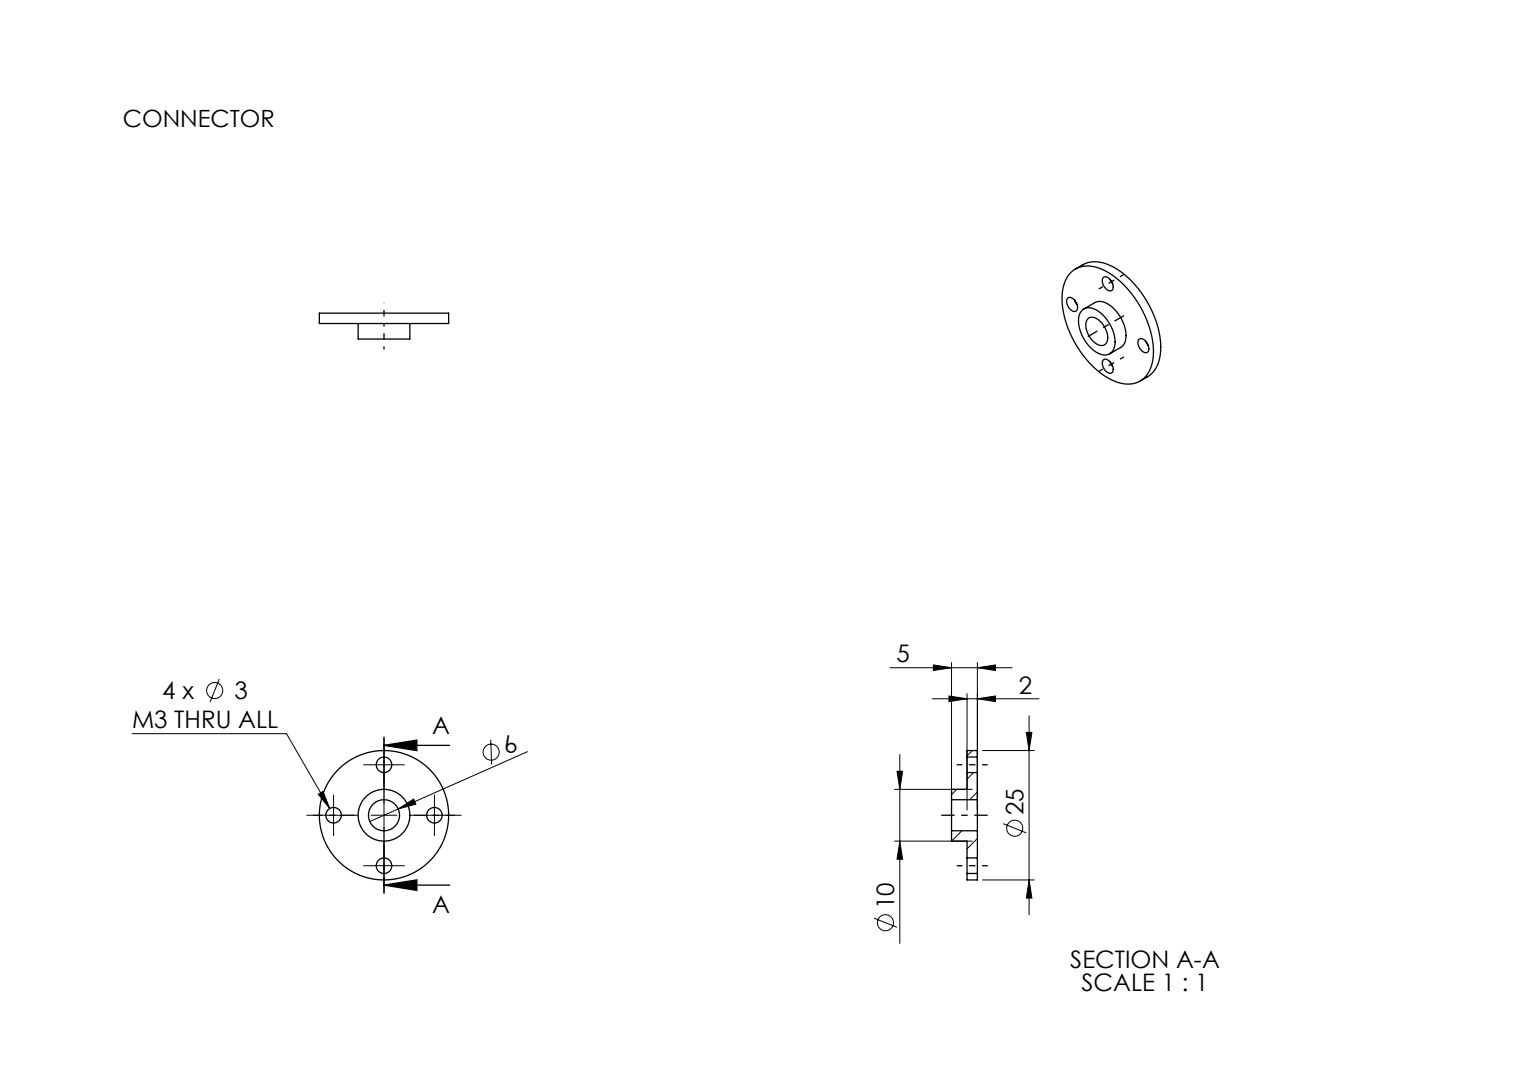
ISO-10303-21;
HEADER;
FILE_DESCRIPTION (('STEP AP214'),
    '1' );
FILE_NAME ('connector.step',
    '2026-10-04T10:31:01',
    ( '' ),
    ( '' ),
    'SwSTEP 2.0',
    'SolidWorks 2026',
    '' );
FILE_SCHEMA (( 'AUTOMOTIVE_DESIGN' ));
ENDSEC;

DATA;
#41=FACE_BOUND ( 'NONE', #6027, .T. ) ;
#54=DIRECTION ( 'NONE',  ( 0.000000000000000000, 0.000000000000000000, 1.000000000000000000 ) ) ;
#65=DIRECTION ( 'NONE',  ( 1.000000000000000000, 0.000000000000000000, 0.000000000000000000 ) ) ;
#67=ORIENTED_EDGE ( 'NONE', *, *, #457, .F. ) ;
#77=LINE ( 'NONE', #5895, #15592 ) ;
#103=EDGE_LOOP ( 'NONE', ( #8397, #1444 ) ) ;
#146=LINE ( 'NONE', #13353, #5536 ) ;
#156=CARTESIAN_POINT ( 'NONE',  ( 12.50000000000000533, 1.530808498934192113E-15, 0.000000000000000000 ) ) ;
#162=ORIENTED_EDGE ( 'NONE', *, *, #10171, .F. ) ;
#176=CARTESIAN_POINT ( 'NONE',  ( 0.000000000000000000, 0.000000000000000000, 5.000000000000004441 ) ) ;
#183=LINE ( 'NONE', #11083, #4538 ) ;
#188=DIRECTION ( 'NONE',  ( 0.000000000000000000, 0.000000000000000000, 1.000000000000000000 ) ) ;
#206=CARTESIAN_POINT ( 'NONE',  ( -12.50000000000000533, 0.000000000000000000, 2.000000000000001776 ) ) ;
#218=DIRECTION ( 'NONE',  ( 0.000000000000000000, 0.000000000000000000, -1.000000000000000000 ) ) ;
#226=EDGE_LOOP ( 'NONE', ( #14083, #11757, #15041, #247 ) ) ;
#228=CARTESIAN_POINT ( 'NONE',  ( -11.25000000000000355, 3.419666426228851687E-14, 2.000000000000001776 ) ) ;
#239=ORIENTED_EDGE ( 'NONE', *, *, #1750, .T. ) ;
#247=ORIENTED_EDGE ( 'NONE', *, *, #524, .F. ) ;
#282=CARTESIAN_POINT ( 'NONE',  ( 1.500000000000000000, -9.750000000000003553, 2.000000000000001776 ) ) ;
#288=( NAMED_UNIT ( * ) SI_UNIT ( $, .STERADIAN. ) SOLID_ANGLE_UNIT ( ) );
#297=CYLINDRICAL_SURFACE ( 'NONE', #14167, 1.499999999999999556 ) ;
#304=DIRECTION ( 'NONE',  ( 0.000000000000000000, 0.000000000000000000, 1.000000000000000000 ) ) ;
#319=DIRECTION ( 'NONE',  ( 1.000000000000000000, 0.000000000000000000, 0.000000000000000000 ) ) ;
#393=DIRECTION ( 'NONE',  ( 1.000000000000000000, 0.000000000000000000, 0.000000000000000000 ) ) ;
#402=DIRECTION ( 'NONE',  ( 1.000000000000000000, 0.000000000000000000, 0.000000000000000000 ) ) ;
#409=DIRECTION ( 'NONE',  ( 1.000000000000000000, 0.000000000000000000, 0.000000000000000000 ) ) ;
#435=DIRECTION ( 'NONE',  ( 0.000000000000000000, 0.000000000000000000, -1.000000000000000000 ) ) ;
#440=LINE ( 'NONE', #9200, #5916 ) ;
#446=AXIS2_PLACEMENT_3D ( 'NONE', #11551, #13858, #6488 ) ;
#457=EDGE_CURVE ( 'NONE', #15709, #6637, #10482, .T. ) ;
#482=CARTESIAN_POINT ( 'NONE',  ( -9.750000000000003553, 3.401296724241641415E-14, 2.000000000000001776 ) ) ;
#486=DIRECTION ( 'NONE',  ( 0.000000000000000000, 0.000000000000000000, 1.000000000000000000 ) ) ;
#495=ORIENTED_EDGE ( 'NONE', *, *, #4351, .F. ) ;
#512=VERTEX_POINT ( 'NONE', #14445 ) ;
#524=EDGE_CURVE ( 'NONE', #8787, #10326, #14889, .T. ) ;
#532=ORIENTED_EDGE ( 'NONE', *, *, #10481, .F. ) ;
#594=EDGE_CURVE ( 'NONE', #12272, #12484, #3857, .T. ) ;
#639=EDGE_CURVE ( 'NONE', #1178, #15136, #14644, .T. ) ;
#670=DIRECTION ( 'NONE',  ( 0.000000000000000000, 0.000000000000000000, 1.000000000000000000 ) ) ;
#775=( LENGTH_UNIT ( ) NAMED_UNIT ( * ) SI_UNIT ( .MILLI., .METRE. ) );
#788=EDGE_CURVE ( 'NONE', #5458, #12720, #7023, .T. ) ;
#816=AXIS2_PLACEMENT_3D ( 'NONE', #2518, #3778, #4670 ) ;
#859=LINE ( 'NONE', #9458, #13806 ) ;
#878=VERTEX_POINT ( 'NONE', #12172 ) ;
#897=MECHANICAL_DESIGN_GEOMETRIC_PRESENTATION_REPRESENTATION('',(#8272),#8792);
#904=UNCERTAINTY_MEASURE_WITH_UNIT (LENGTH_MEASURE( 1.000000000000000082E-05 ), #8679, 'distance_accuracy_value', 'NONE');
#920=VERTEX_POINT ( 'NONE', #156 ) ;
#1053=LINE ( 'NONE', #4803, #11886 ) ;
#1080=AXIS2_PLACEMENT_3D ( 'NONE', #13512, #14641, #13442 ) ;
#1118=ORIENTED_EDGE ( 'NONE', *, *, #11482, .T. ) ;
#1133=VERTEX_POINT ( 'NONE', #11682 ) ;
#1140=FACE_BOUND ( 'NONE', #7178, .T. ) ;
#1145=DIRECTION ( 'NONE',  ( -1.000000000000000000, 0.000000000000000000, 0.000000000000000000 ) ) ;
#1152=DIRECTION ( 'NONE',  ( 1.000000000000000000, 0.000000000000000000, 0.000000000000000000 ) ) ;
#1178=VERTEX_POINT ( 'NONE', #15425 ) ;
#1194=ORIENTED_EDGE ( 'NONE', *, *, #6676, .T. ) ;
#1209=CARTESIAN_POINT ( 'NONE',  ( 12.50000000000000533, 1.530808498934192113E-15, 2.000000000000001776 ) ) ;
#1213=CIRCLE ( 'NONE', #1462, 3.000000000000000000 ) ;
#1248=DIRECTION ( 'NONE',  ( 0.000000000000000000, 0.000000000000000000, 1.000000000000000000 ) ) ;
#1265=CARTESIAN_POINT ( 'NONE',  ( -2.897581130414634077E-17, 9.750000000000003553, 2.000000000000001776 ) ) ;
#1294=DIRECTION ( 'NONE',  ( 0.000000000000000000, 0.000000000000000000, 1.000000000000000000 ) ) ;
#1338=CIRCLE ( 'NONE', #13277, 1.500000000000000000 ) ;
#1378=CARTESIAN_POINT ( 'NONE',  ( 0.000000000000000000, 0.000000000000000000, 2.000000000000001776 ) ) ;
#1432=EDGE_CURVE ( 'NONE', #878, #13950, #13112, .T. ) ;
#1444=ORIENTED_EDGE ( 'NONE', *, *, #13970, .F. ) ;
#1462=AXIS2_PLACEMENT_3D ( 'NONE', #1507, #11295, #393 ) ;
#1468=CARTESIAN_POINT ( 'NONE',  ( 2.897581130414634077E-17, -9.750000000000003553, 2.000000000000001776 ) ) ;
#1507=CARTESIAN_POINT ( 'NONE',  ( 0.000000000000000000, 0.000000000000000000, 5.000000000000004441 ) ) ;
#1511=FACE_OUTER_BOUND ( 'NONE', #12331, .T. ) ;
#1519=ADVANCED_FACE ( 'NONE', ( #3542, #41 ), #8413, .T. ) ;
#1586=ORIENTED_EDGE ( 'NONE', *, *, #13291, .F. ) ;
#1622=ADVANCED_FACE ( 'NONE', ( #14135 ), #15187, .T. ) ;
#1637=AXIS2_PLACEMENT_3D ( 'NONE', #11385, #486, #15285 ) ;
#1651=DIRECTION ( 'NONE',  ( 1.000000000000000000, 0.000000000000000000, 0.000000000000000000 ) ) ;
#1740=ORIENTED_EDGE ( 'NONE', *, *, #8830, .T. ) ;
#1750=EDGE_CURVE ( 'NONE', #2410, #3136, #2201, .T. ) ;
#1778=ORIENTED_EDGE ( 'NONE', *, *, #13016, .T. ) ;
#1814=FACE_OUTER_BOUND ( 'NONE', #10483, .T. ) ;
#1823=ADVANCED_FACE ( 'NONE', ( #12301 ), #7614, .T. ) ;
#1834=CIRCLE ( 'NONE', #816, 1.500000000000000000 ) ;
#1847=CIRCLE ( 'NONE', #2630, 1.499999999999999556 ) ;
#1882=CYLINDRICAL_SURFACE ( 'NONE', #12144, 1.499999999999999556 ) ;
#1887=DIRECTION ( 'NONE',  ( 0.000000000000000000, 0.000000000000000000, -1.000000000000000000 ) ) ;
#1891=DIRECTION ( 'NONE',  ( 0.000000000000000000, 0.000000000000000000, 1.000000000000000000 ) ) ;
#1957=ORIENTED_EDGE ( 'NONE', *, *, #12525, .T. ) ;
#1972=CIRCLE ( 'NONE', #6060, 5.000000000000000000 ) ;
#1974=AXIS2_PLACEMENT_3D ( 'NONE', #8448, #2622, #7478 ) ;
#2004=EDGE_CURVE ( 'NONE', #15509, #10326, #146, .T. ) ;
#2114=ORIENTED_EDGE ( 'NONE', *, *, #11739, .F. ) ;
#2117=DIRECTION ( 'NONE',  ( 0.000000000000000000, 0.000000000000000000, 1.000000000000000000 ) ) ;
#2137=CARTESIAN_POINT ( 'NONE',  ( -5.000000000000000000, 0.000000000000000000, 2.000000000000001776 ) ) ;
#2149=EDGE_CURVE ( 'NONE', #12720, #2410, #13507, .T. ) ;
#2195=EDGE_CURVE ( 'NONE', #9577, #3564, #5089, .T. ) ;
#2201=CIRCLE ( 'NONE', #15686, 1.499999999999999556 ) ;
#2304=CYLINDRICAL_SURFACE ( 'NONE', #13300, 1.500000000000000000 ) ;
#2333=UNCERTAINTY_MEASURE_WITH_UNIT (LENGTH_MEASURE( 1.000000000000000082E-05 ), #8736, 'distance_accuracy_value', 'NONE');
#2352=LINE ( 'NONE', #14611, #7682 ) ;
#2398=CIRCLE ( 'NONE', #5980, 5.000000000000000000 ) ;
#2410=VERTEX_POINT ( 'NONE', #7285 ) ;
#2425=AXIS2_PLACEMENT_3D ( 'NONE', #10542, #15483, #4496 ) ;
#2429=VERTEX_POINT ( 'NONE', #11011 ) ;
#2442=SHAPE_REPRESENTATION_RELATIONSHIP ( 'NONE' , 'NONE' ,  #3660, #4613 ) ;
#2498=EDGE_CURVE ( 'NONE', #3136, #2410, #6811, .T. ) ;
#2504=CYLINDRICAL_SURFACE ( 'NONE', #14010, 3.000000000000000000 ) ;
#2518=CARTESIAN_POINT ( 'NONE',  ( -2.897581130414634077E-17, 9.750000000000003553, 0.000000000000000000 ) ) ;
#2550=CARTESIAN_POINT ( 'NONE',  ( -9.750000000000003553, 3.401296724241641415E-14, 0.000000000000000000 ) ) ;
#2577=DIRECTION ( 'NONE',  ( 0.000000000000000000, 0.000000000000000000, -1.000000000000000000 ) ) ;
#2599=CARTESIAN_POINT ( 'NONE',  ( 0.000000000000000000, 0.000000000000000000, 5.000000000000004441 ) ) ;
#2622=DIRECTION ( 'NONE',  ( 0.000000000000000000, 0.000000000000000000, 1.000000000000000000 ) ) ;
#2630=AXIS2_PLACEMENT_3D ( 'NONE', #6474, #15129, #11308 ) ;
#2651=EDGE_CURVE ( 'NONE', #9577, #15709, #4254, .T. ) ;
#2672=DIRECTION ( 'NONE',  ( 0.000000000000000000, 0.000000000000000000, 1.000000000000000000 ) ) ;
#2747=AXIS2_PLACEMENT_3D ( 'NONE', #6769, #14144, #10650 ) ;
#2770=AXIS2_PLACEMENT_3D ( 'NONE', #176, #10049, #409 ) ;
#2777=FACE_BOUND ( 'NONE', #103, .T. ) ;
#2789=MECHANICAL_DESIGN_GEOMETRIC_PRESENTATION_REPRESENTATION('',(#4319),#14743);
#2919=VECTOR ( 'NONE', #8245, 1000.000000000000000 ) ;
#2952=AXIS2_PLACEMENT_3D ( 'NONE', #2550, #14647, #10822 ) ;
#2974=DIRECTION ( 'NONE',  ( 0.000000000000000000, 0.000000000000000000, 1.000000000000000000 ) ) ;
#3004=AXIS2_PLACEMENT_3D ( 'NONE', #12157, #11913, #65 ) ;
#3039=AXIS2_PLACEMENT_3D ( 'NONE', #6856, #13626, #10063 ) ;
#3044=ORIENTED_EDGE ( 'NONE', *, *, #9648, .F. ) ;
#3074=PRODUCT_DEFINITION_CONTEXT ( 'detailed design', #12070, 'design' ) ;
#3125=FACE_OUTER_BOUND ( 'NONE', #13175, .T. ) ;
#3136=VERTEX_POINT ( 'NONE', #8994 ) ;
#3210=ORIENTED_EDGE ( 'NONE', *, *, #1750, .F. ) ;
#3267=ADVANCED_FACE ( 'NONE', ( #12778 ), #1882, .F. ) ;
#3289=ORIENTED_EDGE ( 'NONE', *, *, #8249, .F. ) ;
#3347=ORIENTED_EDGE ( 'NONE', *, *, #11780, .F. ) ;
#3377=CARTESIAN_POINT ( 'NONE',  ( 12.50000000000000533, 1.530808498934192113E-15, 2.000000000000001776 ) ) ;
#3455=DIRECTION ( 'NONE',  ( 0.000000000000000000, 0.000000000000000000, 1.000000000000000000 ) ) ;
#3542=FACE_OUTER_BOUND ( 'NONE', #14730, .T. ) ;
#3556=COLOUR_RGB ( '', 0.40784314, 0.44705882, 0.49803922) ;
#3564=VERTEX_POINT ( 'NONE', #2137 ) ;
#3585=EDGE_LOOP ( 'NONE', ( #9691, #5379, #12917, #11080 ) ) ;
#3587=ORIENTED_EDGE ( 'NONE', *, *, #7892, .T. ) ;
#3599=ORIENTED_EDGE ( 'NONE', *, *, #2498, .T. ) ;
#3660=SHAPE_REPRESENTATION ( 'connector', ( #14201 ), #13708 ) ;
#3680=ORIENTED_EDGE ( 'NONE', *, *, #788, .F. ) ;
#3706=VECTOR ( 'NONE', #435, 1000.000000000000000 ) ;
#3710=FILL_AREA_STYLE ('',( #11189 ) ) ;
#3721=CARTESIAN_POINT ( 'NONE',  ( 8.250000000000003553, -1.019131563299854308E-13, 2.000000000000001776 ) ) ;
#3750=CARTESIAN_POINT ( 'NONE',  ( 9.750000000000003553, -1.020968533498575335E-13, 0.000000000000000000 ) ) ;
#3767=CARTESIAN_POINT ( 'NONE',  ( 5.000000000000000000, 6.123233995736766282E-16, 2.000000000000001776 ) ) ;
#3778=DIRECTION ( 'NONE',  ( 0.000000000000000000, 0.000000000000000000, 1.000000000000000000 ) ) ;
#3780=DIRECTION ( 'NONE',  ( 0.000000000000000000, 0.000000000000000000, -1.000000000000000000 ) ) ;
#3806=PRESENTATION_STYLE_ASSIGNMENT (( #7165 ) ) ;
#3809=FACE_BOUND ( 'NONE', #5043, .T. ) ;
#3814=ADVANCED_FACE ( 'NONE', ( #13359 ), #7401, .F. ) ;
#3834=ORIENTED_EDGE ( 'NONE', *, *, #11087, .T. ) ;
#3854=ADVANCED_FACE ( 'NONE', ( #12087 ), #11133, .F. ) ;
#3857=LINE ( 'NONE', #206, #3706 ) ;
#3859=CIRCLE ( 'NONE', #5903, 12.50000000000000533 ) ;
#3878=CIRCLE ( 'NONE', #10488, 1.500000000000000000 ) ;
#3882=FACE_BOUND ( 'NONE', #7908, .T. ) ;
#3911=ORIENTED_EDGE ( 'NONE', *, *, #13470, .F. ) ;
#3971=ORIENTED_EDGE ( 'NONE', *, *, #8593, .F. ) ;
#4015=DIRECTION ( 'NONE',  ( 1.000000000000000000, 0.000000000000000000, 0.000000000000000000 ) ) ;
#4146=DIRECTION ( 'NONE',  ( 1.000000000000000000, 0.000000000000000000, 0.000000000000000000 ) ) ;
#4237=EDGE_CURVE ( 'NONE', #7182, #15136, #1053, .T. ) ;
#4254=CIRCLE ( 'NONE', #9097, 5.000000000000000000 ) ;
#4312=AXIS2_PLACEMENT_3D ( 'NONE', #9668, #14509, #7041 ) ;
#4319=STYLED_ITEM ( 'NONE', ( #11033 ), #4613 ) ;
#4322=AXIS2_PLACEMENT_3D ( 'NONE', #10172, #10019, #14866 ) ;
#4334=ORIENTED_EDGE ( 'NONE', *, *, #2149, .T. ) ;
#4351=EDGE_CURVE ( 'NONE', #8237, #15509, #14960, .T. ) ;
#4388=CARTESIAN_POINT ( 'NONE',  ( -2.897581130414634077E-17, 9.750000000000003553, 0.000000000000000000 ) ) ;
#4419=EDGE_LOOP ( 'NONE', ( #8309, #10379, #12079, #7755 ) ) ;
#4474=DIRECTION ( 'NONE',  ( 0.000000000000000000, 0.000000000000000000, -1.000000000000000000 ) ) ;
#4496=DIRECTION ( 'NONE',  ( 1.000000000000000000, 0.000000000000000000, 0.000000000000000000 ) ) ;
#4538=VECTOR ( 'NONE', #1294, 1000.000000000000000 ) ;
#4567=CARTESIAN_POINT ( 'NONE',  ( -12.50000000000000533, 0.000000000000000000, 2.000000000000001776 ) ) ;
#4613=ADVANCED_BREP_SHAPE_REPRESENTATION ( '', ( #10345, #14201 ), #13708 ) ;
#4614=CARTESIAN_POINT ( 'NONE',  ( 0.000000000000000000, 0.000000000000000000, 5.000000000000004441 ) ) ;
#4634=CARTESIAN_POINT ( 'NONE',  ( 0.000000000000000000, 0.000000000000000000, 5.000000000000004441 ) ) ;
#4667=CARTESIAN_POINT ( 'NONE',  ( -11.25000000000000355, 3.419666426228851687E-14, 0.000000000000000000 ) ) ;
#4670=DIRECTION ( 'NONE',  ( 1.000000000000000000, 0.000000000000000000, 0.000000000000000000 ) ) ;
#4727=EDGE_LOOP ( 'NONE', ( #6809, #1118 ) ) ;
#4738=CARTESIAN_POINT ( 'NONE',  ( 0.000000000000000000, 0.000000000000000000, 2.000000000000001776 ) ) ;
#4771=PRODUCT_DEFINITION_FORMATION_WITH_SPECIFIED_SOURCE ( 'ANY', '', #12844, .NOT_KNOWN. ) ;
#4803=CARTESIAN_POINT ( 'NONE',  ( 1.500000000000000000, -9.750000000000003553, 2.000000000000001776 ) ) ;
#4813=PLANE ( 'NONE',  #4312 ) ;
#4840=SURFACE_STYLE_FILL_AREA ( #3710 ) ;
#4849=ADVANCED_FACE ( 'NONE', ( #8400, #1140, #4894, #6005, #1511, #10848 ), #4813, .F. ) ;
#4858=FILL_AREA_STYLE ('',( #13278 ) ) ;
#4894=FACE_BOUND ( 'NONE', #4727, .T. ) ;
#4910=ORIENTED_EDGE ( 'NONE', *, *, #8830, .F. ) ;
#4913=DIRECTION ( 'NONE',  ( 0.000000000000000000, 0.000000000000000000, 1.000000000000000000 ) ) ;
#5003=ORIENTED_EDGE ( 'NONE', *, *, #8249, .T. ) ;
#5022=ORIENTED_EDGE ( 'NONE', *, *, #594, .T. ) ;
#5043=EDGE_LOOP ( 'NONE', ( #14358, #3210 ) ) ;
#5089=LINE ( 'NONE', #10174, #11620 ) ;
#5197=ORIENTED_EDGE ( 'NONE', *, *, #10481, .T. ) ;
#5221=EDGE_CURVE ( 'NONE', #8237, #8787, #8440, .T. ) ;
#5315=LINE ( 'NONE', #11420, #7927 ) ;
#5340=EDGE_LOOP ( 'NONE', ( #4910, #5511, #14806, #14609 ) ) ;
#5372=ADVANCED_FACE ( 'NONE', ( #6447 ), #15178, .F. ) ;
#5379=ORIENTED_EDGE ( 'NONE', *, *, #14202, .T. ) ;
#5458=VERTEX_POINT ( 'NONE', #7932 ) ;
#5460=CIRCLE ( 'NONE', #5707, 1.499999999999999556 ) ;
#5493=DIRECTION ( 'NONE',  ( 0.000000000000000000, 0.000000000000000000, -1.000000000000000000 ) ) ;
#5511=ORIENTED_EDGE ( 'NONE', *, *, #7181, .F. ) ;
#5536=VECTOR ( 'NONE', #15673, 1000.000000000000000 ) ;
#5558=ORIENTED_EDGE ( 'NONE', *, *, #5221, .T. ) ;
#5676=CARTESIAN_POINT ( 'NONE',  ( 0.000000000000000000, 0.000000000000000000, 2.000000000000001776 ) ) ;
#5707=AXIS2_PLACEMENT_3D ( 'NONE', #12298, #54, #9776 ) ;
#5727=ORIENTED_EDGE ( 'NONE', *, *, #7781, .T. ) ;
#5738=AXIS2_PLACEMENT_3D ( 'NONE', #8418, #4913, #7447 ) ;
#5838=DIRECTION ( 'NONE',  ( 0.000000000000000000, 0.000000000000000000, 1.000000000000000000 ) ) ;
#5881=CARTESIAN_POINT ( 'NONE',  ( -5.000000000000000000, 0.000000000000000000, 5.000000000000004441 ) ) ;
#5895=CARTESIAN_POINT ( 'NONE',  ( -1.500000000000000000, 9.750000000000003553, 2.000000000000001776 ) ) ;
#5903=AXIS2_PLACEMENT_3D ( 'NONE', #1378, #188, #14431 ) ;
#5916=VECTOR ( 'NONE', #670, 1000.000000000000000 ) ;
#5980=AXIS2_PLACEMENT_3D ( 'NONE', #4614, #9549, #13111 ) ;
#6005=FACE_BOUND ( 'NONE', #7392, .T. ) ;
#6023=ORIENTED_EDGE ( 'NONE', *, *, #4237, .T. ) ;
#6027=EDGE_LOOP ( 'NONE', ( #15025, #495 ) ) ;
#6060=AXIS2_PLACEMENT_3D ( 'NONE', #14965, #9956, #319 ) ;
#6063=DIRECTION ( 'NONE',  ( 0.000000000000000000, 0.000000000000000000, 1.000000000000000000 ) ) ;
#6123=DIRECTION ( 'NONE',  ( 1.000000000000000000, 0.000000000000000000, 0.000000000000000000 ) ) ;
#6136=CARTESIAN_POINT ( 'NONE',  ( -3.000000000000000000, 0.000000000000000000, 0.000000000000000000 ) ) ;
#6151=EDGE_LOOP ( 'NONE', ( #9273, #1194 ) ) ;
#6214=SURFACE_SIDE_STYLE ('',( #11128 ) ) ;
#6227=AXIS2_PLACEMENT_3D ( 'NONE', #9435, #9280, #14267 ) ;
#6290=FACE_OUTER_BOUND ( 'NONE', #6151, .T. ) ;
#6407=ORIENTED_EDGE ( 'NONE', *, *, #2149, .F. ) ;
#6442=DIRECTION ( 'NONE',  ( 0.000000000000000000, 0.000000000000000000, 1.000000000000000000 ) ) ;
#6447=FACE_OUTER_BOUND ( 'NONE', #3585, .T. ) ;
#6474=CARTESIAN_POINT ( 'NONE',  ( 9.750000000000003553, -1.020968533498575335E-13, 2.000000000000001776 ) ) ;
#6488=DIRECTION ( 'NONE',  ( 1.000000000000000000, 0.000000000000000000, 0.000000000000000000 ) ) ;
#6518=DIRECTION ( 'NONE',  ( 1.000000000000000000, 0.000000000000000000, 0.000000000000000000 ) ) ;
#6599=ADVANCED_FACE ( 'NONE', ( #10936 ), #2504, .F. ) ;
#6637=VERTEX_POINT ( 'NONE', #3767 ) ;
#6651=ADVANCED_FACE ( 'NONE', ( #13475 ), #10778, .T. ) ;
#6676=EDGE_CURVE ( 'NONE', #12347, #12272, #3859, .T. ) ;
#6680=CARTESIAN_POINT ( 'NONE',  ( 0.000000000000000000, 0.000000000000000000, 0.000000000000000000 ) ) ;
#6693=AXIS2_PLACEMENT_3D ( 'NONE', #3750, #8701, #13534 ) ;
#6705=DIRECTION ( 'NONE',  ( 0.000000000000000000, 0.000000000000000000, 1.000000000000000000 ) ) ;
#6722=CARTESIAN_POINT ( 'NONE',  ( 2.897581130414634077E-17, -9.750000000000003553, 2.000000000000001776 ) ) ;
#6757=DIRECTION ( 'NONE',  ( 1.000000000000000000, 0.000000000000000000, 0.000000000000000000 ) ) ;
#6769=CARTESIAN_POINT ( 'NONE',  ( 0.000000000000000000, 0.000000000000000000, 0.000000000000000000 ) ) ;
#6774=AXIS2_PLACEMENT_3D ( 'NONE', #1468, #2672, #4015 ) ;
#6780=CARTESIAN_POINT ( 'NONE',  ( 3.000000000000000000, 3.673940397442059868E-16, 0.000000000000000000 ) ) ;
#6806=ORIENTED_EDGE ( 'NONE', *, *, #7218, .T. ) ;
#6809=ORIENTED_EDGE ( 'NONE', *, *, #8294, .T. ) ;
#6811=CIRCLE ( 'NONE', #446, 1.499999999999999556 ) ;
#6823=AXIS2_PLACEMENT_3D ( 'NONE', #1265, #9637, #12322 ) ;
#6825=CARTESIAN_POINT ( 'NONE',  ( -2.897581130414634077E-17, 9.750000000000003553, 2.000000000000001776 ) ) ;
#6826=ADVANCED_FACE ( 'NONE', ( #9013 ), #10197, .F. ) ;
#6856=CARTESIAN_POINT ( 'NONE',  ( -2.897581130414634077E-17, 9.750000000000003553, 2.000000000000001776 ) ) ;
#6904=DIRECTION ( 'NONE',  ( 1.000000000000000000, 0.000000000000000000, 0.000000000000000000 ) ) ;
#6943=ORIENTED_EDGE ( 'NONE', *, *, #788, .T. ) ;
#6951=CYLINDRICAL_SURFACE ( 'NONE', #11523, 3.000000000000000000 ) ;
#6981=CIRCLE ( 'NONE', #6227, 1.500000000000000000 ) ;
#7023=CIRCLE ( 'NONE', #2952, 1.499999999999999556 ) ;
#7041=DIRECTION ( 'NONE',  ( 1.000000000000000000, 0.000000000000000000, 0.000000000000000000 ) ) ;
#7081=ADVANCED_FACE ( 'NONE', ( #8202, #2777, #14721, #3809, #6290, #3882 ), #8682, .T. ) ;
#7115=ORIENTED_EDGE ( 'NONE', *, *, #11087, .F. ) ;
#7119=ORIENTED_EDGE ( 'NONE', *, *, #8294, .F. ) ;
#7165=SURFACE_STYLE_USAGE ( .BOTH. , #6214 ) ;
#7178=EDGE_LOOP ( 'NONE', ( #12111, #3834 ) ) ;
#7181=EDGE_CURVE ( 'NONE', #10893, #512, #1834, .T. ) ;
#7182=VERTEX_POINT ( 'NONE', #11892 ) ;
#7199=ORIENTED_EDGE ( 'NONE', *, *, #2651, .T. ) ;
#7218=EDGE_CURVE ( 'NONE', #2429, #13435, #2352, .T. ) ;
#7277=EDGE_LOOP ( 'NONE', ( #3289, #14486 ) ) ;
#7285=CARTESIAN_POINT ( 'NONE',  ( -11.25000000000000355, 3.419666426228851687E-14, 2.000000000000001776 ) ) ;
#7305=SURFACE_STYLE_USAGE ( .BOTH. , #9925 ) ;
#7309=CARTESIAN_POINT ( 'NONE',  ( -9.750000000000003553, 3.401296724241641415E-14, 2.000000000000001776 ) ) ;
#7392=EDGE_LOOP ( 'NONE', ( #6943, #8269 ) ) ;
#7401=CYLINDRICAL_SURFACE ( 'NONE', #6823, 1.500000000000000000 ) ;
#7411=ORIENTED_EDGE ( 'NONE', *, *, #594, .F. ) ;
#7426=ORIENTED_EDGE ( 'NONE', *, *, #2195, .T. ) ;
#7434=CARTESIAN_POINT ( 'NONE',  ( 0.000000000000000000, 0.000000000000000000, 5.000000000000004441 ) ) ;
#7445=DIRECTION ( 'NONE',  ( 0.000000000000000000, 0.000000000000000000, 1.000000000000000000 ) ) ;
#7447=DIRECTION ( 'NONE',  ( 1.000000000000000000, 0.000000000000000000, 0.000000000000000000 ) ) ;
#7478=DIRECTION ( 'NONE',  ( 1.000000000000000000, 0.000000000000000000, 0.000000000000000000 ) ) ;
#7486=EDGE_LOOP ( 'NONE', ( #14634, #15623 ) ) ;
#7614=CYLINDRICAL_SURFACE ( 'NONE', #8062, 5.000000000000000000 ) ;
#7624=ORIENTED_EDGE ( 'NONE', *, *, #8678, .T. ) ;
#7682=VECTOR ( 'NONE', #14689, 1000.000000000000000 ) ;
#7755=ORIENTED_EDGE ( 'NONE', *, *, #2195, .F. ) ;
#7756=CARTESIAN_POINT ( 'NONE',  ( -1.500000000000000000, 9.750000000000003553, 2.000000000000001776 ) ) ;
#7767=CIRCLE ( 'NONE', #2425, 3.000000000000000000 ) ;
#7781=EDGE_CURVE ( 'NONE', #5458, #3136, #440, .T. ) ;
#7791=ORIENTED_EDGE ( 'NONE', *, *, #13123, .T. ) ;
#7851=EDGE_CURVE ( 'NONE', #8910, #1133, #5315, .T. ) ;
#7892=EDGE_CURVE ( 'NONE', #920, #12484, #12002, .T. ) ;
#7908=EDGE_LOOP ( 'NONE', ( #10647, #3911 ) ) ;
#7927=VECTOR ( 'NONE', #10160, 1000.000000000000000 ) ;
#7932=CARTESIAN_POINT ( 'NONE',  ( -8.250000000000003553, 3.401296724241641415E-14, 0.000000000000000000 ) ) ;
#8040=CYLINDRICAL_SURFACE ( 'NONE', #3039, 1.500000000000000000 ) ;
#8049=EDGE_LOOP ( 'NONE', ( #9978, #7119, #6023, #5003 ) ) ;
#8062=AXIS2_PLACEMENT_3D ( 'NONE', #2599, #218, #13496 ) ;
#8202=FACE_BOUND ( 'NONE', #14381, .T. ) ;
#8237=VERTEX_POINT ( 'NONE', #13862 ) ;
#8245=DIRECTION ( 'NONE',  ( 0.000000000000000000, 0.000000000000000000, -1.000000000000000000 ) ) ;
#8249=EDGE_CURVE ( 'NONE', #15136, #1178, #3878, .T. ) ;
#8269=ORIENTED_EDGE ( 'NONE', *, *, #10673, .T. ) ;
#8272=STYLED_ITEM ( 'NONE', ( #3806 ), #10345 ) ;
#8294=EDGE_CURVE ( 'NONE', #7182, #14655, #1338, .T. ) ;
#8309=ORIENTED_EDGE ( 'NONE', *, *, #12525, .F. ) ;
#8333=EDGE_LOOP ( 'NONE', ( #15336, #4334, #239, #15665 ) ) ;
#8354=AXIS2_PLACEMENT_3D ( 'NONE', #9997, #7445, #12289 ) ;
#8397=ORIENTED_EDGE ( 'NONE', *, *, #8678, .F. ) ;
#8400=FACE_BOUND ( 'NONE', #7486, .T. ) ;
#8404=UNCERTAINTY_MEASURE_WITH_UNIT (LENGTH_MEASURE( 1.000000000000000082E-05 ), #775, 'distance_accuracy_value', 'NONE');
#8413=PLANE ( 'NONE',  #14136 ) ;
#8418=CARTESIAN_POINT ( 'NONE',  ( 0.000000000000000000, 0.000000000000000000, 0.000000000000000000 ) ) ;
#8440=LINE ( 'NONE', #9711, #12943 ) ;
#8448=CARTESIAN_POINT ( 'NONE',  ( 9.750000000000003553, -1.020968533498575335E-13, 2.000000000000001776 ) ) ;
#8458=AXIS2_PLACEMENT_3D ( 'NONE', #482, #11380, #402 ) ;
#8509=( NAMED_UNIT ( * ) PLANE_ANGLE_UNIT ( ) SI_UNIT ( $, .RADIAN. ) );
#8522=CIRCLE ( 'NONE', #1637, 1.500000000000000000 ) ;
#8593=EDGE_CURVE ( 'NONE', #8910, #2429, #11502, .T. ) ;
#8678=EDGE_CURVE ( 'NONE', #1133, #13435, #1847, .T. ) ;
#8679=( LENGTH_UNIT ( ) NAMED_UNIT ( * ) SI_UNIT ( .MILLI., .METRE. ) );
#8682=PLANE ( 'NONE',  #1080 ) ;
#8701=DIRECTION ( 'NONE',  ( 0.000000000000000000, 0.000000000000000000, 1.000000000000000000 ) ) ;
#8736=( LENGTH_UNIT ( ) NAMED_UNIT ( * ) SI_UNIT ( .MILLI., .METRE. ) );
#8749=AXIS2_PLACEMENT_3D ( 'NONE', #8761, #5493, #13594 ) ;
#8761=CARTESIAN_POINT ( 'NONE',  ( 0.000000000000000000, 0.000000000000000000, 5.000000000000004441 ) ) ;
#8769=EDGE_LOOP ( 'NONE', ( #7115, #6806, #11599, #10192 ) ) ;
#8787=VERTEX_POINT ( 'NONE', #6780 ) ;
#8792=( GEOMETRIC_REPRESENTATION_CONTEXT ( 3 ) GLOBAL_UNCERTAINTY_ASSIGNED_CONTEXT ( ( #904 ) ) GLOBAL_UNIT_ASSIGNED_CONTEXT ( ( #8679, #12317, #12082 ) ) REPRESENTATION_CONTEXT ( 'NONE', 'WORKASPACE' ) );
#8797=FACE_OUTER_BOUND ( 'NONE', #15211, .T. ) ;
#8830=EDGE_CURVE ( 'NONE', #512, #13950, #77, .T. ) ;
#8910=VERTEX_POINT ( 'NONE', #14726 ) ;
#8993=DIRECTION ( 'NONE',  ( 0.000000000000000000, 0.000000000000000000, -1.000000000000000000 ) ) ;
#8994=CARTESIAN_POINT ( 'NONE',  ( -8.250000000000003553, 3.401296724241641415E-14, 2.000000000000001776 ) ) ;
#9007=ORIENTED_EDGE ( 'NONE', *, *, #11780, .T. ) ;
#9013=FACE_OUTER_BOUND ( 'NONE', #8333, .T. ) ;
#9097=AXIS2_PLACEMENT_3D ( 'NONE', #14657, #9807, #9651 ) ;
#9200=CARTESIAN_POINT ( 'NONE',  ( -8.250000000000003553, 3.401296724241641415E-14, 2.000000000000001776 ) ) ;
#9224=CARTESIAN_POINT ( 'NONE',  ( 0.000000000000000000, 0.000000000000000000, 2.000000000000001776 ) ) ;
#9273=ORIENTED_EDGE ( 'NONE', *, *, #10171, .T. ) ;
#9280=DIRECTION ( 'NONE',  ( 0.000000000000000000, 0.000000000000000000, 1.000000000000000000 ) ) ;
#9294=CARTESIAN_POINT ( 'NONE',  ( 1.500000000000000000, 9.750000000000003553, 0.000000000000000000 ) ) ;
#9328=DIRECTION ( 'NONE',  ( -1.000000000000000000, 0.000000000000000000, 0.000000000000000000 ) ) ;
#9338=ADVANCED_FACE ( 'NONE', ( #11058 ), #2304, .F. ) ;
#9366=ORIENTED_EDGE ( 'NONE', *, *, #7892, .F. ) ;
#9435=CARTESIAN_POINT ( 'NONE',  ( 2.897581130414634077E-17, -9.750000000000003553, 0.000000000000000000 ) ) ;
#9458=CARTESIAN_POINT ( 'NONE',  ( 1.500000000000000000, 9.750000000000003553, 2.000000000000001776 ) ) ;
#9461=ADVANCED_FACE ( 'NONE', ( #1814 ), #10105, .T. ) ;
#9549=DIRECTION ( 'NONE',  ( 0.000000000000000000, 0.000000000000000000, 1.000000000000000000 ) ) ;
#9577=VERTEX_POINT ( 'NONE', #5881 ) ;
#9637=DIRECTION ( 'NONE',  ( 0.000000000000000000, 0.000000000000000000, 1.000000000000000000 ) ) ;
#9645=APPLICATION_CONTEXT ( 'automotive_design' ) ;
#9648=EDGE_CURVE ( 'NONE', #10893, #878, #859, .T. ) ;
#9651=DIRECTION ( 'NONE',  ( 1.000000000000000000, 0.000000000000000000, 0.000000000000000000 ) ) ;
#9663=ORIENTED_EDGE ( 'NONE', *, *, #524, .T. ) ;
#9668=CARTESIAN_POINT ( 'NONE',  ( 0.000000000000000000, 0.000000000000000000, 0.000000000000000000 ) ) ;
#9675=DIRECTION ( 'NONE',  ( 0.000000000000000000, 0.000000000000000000, -1.000000000000000000 ) ) ;
#9691=ORIENTED_EDGE ( 'NONE', *, *, #11482, .F. ) ;
#9697=( NAMED_UNIT ( * ) PLANE_ANGLE_UNIT ( ) SI_UNIT ( $, .RADIAN. ) );
#9711=CARTESIAN_POINT ( 'NONE',  ( 3.000000000000000000, 3.673940397442059868E-16, 5.000000000000004441 ) ) ;
#9776=DIRECTION ( 'NONE',  ( 1.000000000000000000, 0.000000000000000000, 0.000000000000000000 ) ) ;
#9804=CARTESIAN_POINT ( 'NONE',  ( -1.500000000000000000, -9.750000000000003553, 0.000000000000000000 ) ) ;
#9807=DIRECTION ( 'NONE',  ( 0.000000000000000000, 0.000000000000000000, 1.000000000000000000 ) ) ;
#9876=CARTESIAN_POINT ( 'NONE',  ( 2.897581130414634077E-17, -9.750000000000003553, 2.000000000000001776 ) ) ;
#9925=SURFACE_SIDE_STYLE ('',( #4840 ) ) ;
#9956=DIRECTION ( 'NONE',  ( 0.000000000000000000, 0.000000000000000000, 1.000000000000000000 ) ) ;
#9957=EDGE_LOOP ( 'NONE', ( #10149, #162, #5022, #10281 ) ) ;
#9973=EDGE_LOOP ( 'NONE', ( #5197, #9663 ) ) ;
#9978=ORIENTED_EDGE ( 'NONE', *, *, #14202, .F. ) ;
#9997=CARTESIAN_POINT ( 'NONE',  ( 9.750000000000003553, -1.020968533498575335E-13, 2.000000000000001776 ) ) ;
#10019=DIRECTION ( 'NONE',  ( 0.000000000000000000, 0.000000000000000000, 1.000000000000000000 ) ) ;
#10049=DIRECTION ( 'NONE',  ( 0.000000000000000000, 0.000000000000000000, 1.000000000000000000 ) ) ;
#10057=AXIS2_PLACEMENT_3D ( 'NONE', #13395, #11090, #12203 ) ;
#10063=DIRECTION ( 'NONE',  ( 1.000000000000000000, 0.000000000000000000, 0.000000000000000000 ) ) ;
#10088=FACE_OUTER_BOUND ( 'NONE', #11279, .T. ) ;
#10105=CYLINDRICAL_SURFACE ( 'NONE', #8749, 5.000000000000000000 ) ;
#10149=ORIENTED_EDGE ( 'NONE', *, *, #11511, .F. ) ;
#10160=DIRECTION ( 'NONE',  ( 0.000000000000000000, 0.000000000000000000, 1.000000000000000000 ) ) ;
#10171=EDGE_CURVE ( 'NONE', #12272, #12347, #10263, .T. ) ;
#10172=CARTESIAN_POINT ( 'NONE',  ( 2.897581130414634077E-17, -9.750000000000003553, 2.000000000000001776 ) ) ;
#10174=CARTESIAN_POINT ( 'NONE',  ( -5.000000000000000000, 0.000000000000000000, 5.000000000000004441 ) ) ;
#10192=ORIENTED_EDGE ( 'NONE', *, *, #7851, .F. ) ;
#10197=CYLINDRICAL_SURFACE ( 'NONE', #8458, 1.499999999999999556 ) ;
#10212=ADVANCED_FACE ( 'NONE', ( #3125 ), #6951, .F. ) ;
#10254=CARTESIAN_POINT ( 'NONE',  ( 5.000000000000000000, 6.123233995736766282E-16, 5.000000000000004441 ) ) ;
#10263=CIRCLE ( 'NONE', #12286, 12.50000000000000533 ) ;
#10281=ORIENTED_EDGE ( 'NONE', *, *, #13291, .T. ) ;
#10290=AXIS2_PLACEMENT_3D ( 'NONE', #4388, #6705, #4146 ) ;
#10326=VERTEX_POINT ( 'NONE', #6136 ) ;
#10345=MANIFOLD_SOLID_BREP ( 'Extrude-Thin1', #14349 ) ;
#10379=ORIENTED_EDGE ( 'NONE', *, *, #457, .T. ) ;
#10481=EDGE_CURVE ( 'NONE', #10326, #8787, #7767, .T. ) ;
#10482=LINE ( 'NONE', #15335, #12335 ) ;
#10483=EDGE_LOOP ( 'NONE', ( #67, #13332, #7426, #1778 ) ) ;
#10488=AXIS2_PLACEMENT_3D ( 'NONE', #6722, #2974, #11556 ) ;
#10524=DIRECTION ( 'NONE',  ( 0.000000000000000000, 0.000000000000000000, 1.000000000000000000 ) ) ;
#10542=CARTESIAN_POINT ( 'NONE',  ( 0.000000000000000000, 0.000000000000000000, 0.000000000000000000 ) ) ;
#10544=DIRECTION ( 'NONE',  ( 1.000000000000000000, 0.000000000000000000, 0.000000000000000000 ) ) ;
#10647=ORIENTED_EDGE ( 'NONE', *, *, #13016, .F. ) ;
#10650=DIRECTION ( 'NONE',  ( 1.000000000000000000, 0.000000000000000000, 0.000000000000000000 ) ) ;
#10673=EDGE_CURVE ( 'NONE', #12720, #5458, #15130, .T. ) ;
#10681=CARTESIAN_POINT ( 'NONE',  ( 2.897581130414634077E-17, -9.750000000000003553, 0.000000000000000000 ) ) ;
#10778=CYLINDRICAL_SURFACE ( 'NONE', #12242, 12.50000000000000533 ) ;
#10822=DIRECTION ( 'NONE',  ( 1.000000000000000000, 0.000000000000000000, 0.000000000000000000 ) ) ;
#10848=FACE_BOUND ( 'NONE', #9973, .T. ) ;
#10893=VERTEX_POINT ( 'NONE', #9294 ) ;
#10908=ORIENTED_EDGE ( 'NONE', *, *, #1432, .F. ) ;
#10936=FACE_OUTER_BOUND ( 'NONE', #226, .T. ) ;
#10982=DIRECTION ( 'NONE',  ( 1.000000000000000000, 0.000000000000000000, 0.000000000000000000 ) ) ;
#11011=CARTESIAN_POINT ( 'NONE',  ( 8.250000000000003553, -1.019131563299854308E-13, 0.000000000000000000 ) ) ;
#11033=PRESENTATION_STYLE_ASSIGNMENT (( #7305 ) ) ;
#11058=FACE_OUTER_BOUND ( 'NONE', #8049, .T. ) ;
#11080=ORIENTED_EDGE ( 'NONE', *, *, #4237, .F. ) ;
#11083=CARTESIAN_POINT ( 'NONE',  ( -1.500000000000000000, -9.750000000000003553, 2.000000000000001776 ) ) ;
#11087=EDGE_CURVE ( 'NONE', #2429, #8910, #5460, .T. ) ;
#11090=DIRECTION ( 'NONE',  ( 0.000000000000000000, 0.000000000000000000, 1.000000000000000000 ) ) ;
#11128=SURFACE_STYLE_FILL_AREA ( #4858 ) ;
#11133=CYLINDRICAL_SURFACE ( 'NONE', #1974, 1.499999999999999556 ) ;
#11189=FILL_AREA_STYLE_COLOUR ( '', #3556 ) ;
#11247=AXIS2_PLACEMENT_3D ( 'NONE', #11882, #3455, #10544 ) ;
#11279=EDGE_LOOP ( 'NONE', ( #15102, #3971, #14102, #7624 ) ) ;
#11295=DIRECTION ( 'NONE',  ( 0.000000000000000000, 0.000000000000000000, 1.000000000000000000 ) ) ;
#11296=CIRCLE ( 'NONE', #10290, 1.500000000000000000 ) ;
#11308=DIRECTION ( 'NONE',  ( 1.000000000000000000, 0.000000000000000000, 0.000000000000000000 ) ) ;
#11359=AXIS2_PLACEMENT_3D ( 'NONE', #9224, #1887, #12783 ) ;
#11380=DIRECTION ( 'NONE',  ( 0.000000000000000000, 0.000000000000000000, 1.000000000000000000 ) ) ;
#11385=CARTESIAN_POINT ( 'NONE',  ( -2.897581130414634077E-17, 9.750000000000003553, 2.000000000000001776 ) ) ;
#11420=CARTESIAN_POINT ( 'NONE',  ( 11.25000000000000355, -1.020968533498575335E-13, 2.000000000000001776 ) ) ;
#11482=EDGE_CURVE ( 'NONE', #14655, #7182, #6981, .T. ) ;
#11502=CIRCLE ( 'NONE', #6693, 1.499999999999999556 ) ;
#11511=EDGE_CURVE ( 'NONE', #12347, #920, #14117, .T. ) ;
#11513=DIRECTION ( 'NONE',  ( 0.000000000000000000, 0.000000000000000000, 1.000000000000000000 ) ) ;
#11523=AXIS2_PLACEMENT_3D ( 'NONE', #4634, #4474, #9328 ) ;
#11551=CARTESIAN_POINT ( 'NONE',  ( -9.750000000000003553, 3.401296724241641415E-14, 2.000000000000001776 ) ) ;
#11556=DIRECTION ( 'NONE',  ( 1.000000000000000000, 0.000000000000000000, 0.000000000000000000 ) ) ;
#11599=ORIENTED_EDGE ( 'NONE', *, *, #13970, .T. ) ;
#11620=VECTOR ( 'NONE', #8993, 1000.000000000000000 ) ;
#11661=DIRECTION ( 'NONE',  ( 0.000000000000000000, 0.000000000000000000, 1.000000000000000000 ) ) ;
#11682=CARTESIAN_POINT ( 'NONE',  ( 11.25000000000000355, -1.020968533498575335E-13, 2.000000000000001776 ) ) ;
#11713=SHAPE_DEFINITION_REPRESENTATION ( #13501, #3660 ) ;
#11739=EDGE_CURVE ( 'NONE', #512, #10893, #11296, .T. ) ;
#11757=ORIENTED_EDGE ( 'NONE', *, *, #4351, .T. ) ;
#11780=EDGE_CURVE ( 'NONE', #13950, #878, #8522, .T. ) ;
#11855=DIRECTION ( 'NONE',  ( 1.000000000000000000, 0.000000000000000000, 0.000000000000000000 ) ) ;
#11882=CARTESIAN_POINT ( 'NONE',  ( 0.000000000000000000, 0.000000000000000000, 0.000000000000000000 ) ) ;
#11886=VECTOR ( 'NONE', #5838, 1000.000000000000000 ) ;
#11892=CARTESIAN_POINT ( 'NONE',  ( 1.500000000000000000, -9.750000000000003553, 0.000000000000000000 ) ) ;
#11913=DIRECTION ( 'NONE',  ( 0.000000000000000000, 0.000000000000000000, 1.000000000000000000 ) ) ;
#12002=CIRCLE ( 'NONE', #11247, 12.50000000000000533 ) ;
#12053=DIRECTION ( 'NONE',  ( 0.000000000000000000, 0.000000000000000000, 1.000000000000000000 ) ) ;
#12070=APPLICATION_CONTEXT ( 'automotive_design' ) ;
#12079=ORIENTED_EDGE ( 'NONE', *, *, #13470, .T. ) ;
#12082=( NAMED_UNIT ( * ) SI_UNIT ( $, .STERADIAN. ) SOLID_ANGLE_UNIT ( ) );
#12087=FACE_OUTER_BOUND ( 'NONE', #8769, .T. ) ;
#12111=ORIENTED_EDGE ( 'NONE', *, *, #8593, .T. ) ;
#12144=AXIS2_PLACEMENT_3D ( 'NONE', #15339, #2117, #6757 ) ;
#12157=CARTESIAN_POINT ( 'NONE',  ( 0.000000000000000000, 0.000000000000000000, 2.000000000000001776 ) ) ;
#12172=CARTESIAN_POINT ( 'NONE',  ( 1.500000000000000000, 9.750000000000003553, 2.000000000000001776 ) ) ;
#12203=DIRECTION ( 'NONE',  ( 1.000000000000000000, 0.000000000000000000, 0.000000000000000000 ) ) ;
#12242=AXIS2_PLACEMENT_3D ( 'NONE', #4738, #2577, #12279 ) ;
#12272=VERTEX_POINT ( 'NONE', #4567 ) ;
#12279=DIRECTION ( 'NONE',  ( -1.000000000000000000, 0.000000000000000000, 0.000000000000000000 ) ) ;
#12286=AXIS2_PLACEMENT_3D ( 'NONE', #5676, #10524, #11855 ) ;
#12289=DIRECTION ( 'NONE',  ( 1.000000000000000000, 0.000000000000000000, 0.000000000000000000 ) ) ;
#12298=CARTESIAN_POINT ( 'NONE',  ( 9.750000000000003553, -1.020968533498575335E-13, 0.000000000000000000 ) ) ;
#12301=FACE_OUTER_BOUND ( 'NONE', #4419, .T. ) ;
#12317=( NAMED_UNIT ( * ) PLANE_ANGLE_UNIT ( ) SI_UNIT ( $, .RADIAN. ) );
#12322=DIRECTION ( 'NONE',  ( 1.000000000000000000, 0.000000000000000000, 0.000000000000000000 ) ) ;
#12331=EDGE_LOOP ( 'NONE', ( #1586, #9366 ) ) ;
#12335=VECTOR ( 'NONE', #3780, 1000.000000000000000 ) ;
#12347=VERTEX_POINT ( 'NONE', #1209 ) ;
#12384=CARTESIAN_POINT ( 'NONE',  ( 9.750000000000003553, -1.020968533498575335E-13, 2.000000000000001776 ) ) ;
#12484=VERTEX_POINT ( 'NONE', #13306 ) ;
#12525=EDGE_CURVE ( 'NONE', #15709, #9577, #2398, .T. ) ;
#12537=COLOUR_RGB ( '', 0.40784314, 0.44705882, 0.49803922) ;
#12644=ADVANCED_FACE ( 'NONE', ( #10088 ), #297, .F. ) ;
#12720=VERTEX_POINT ( 'NONE', #4667 ) ;
#12778=FACE_OUTER_BOUND ( 'NONE', #13600, .T. ) ;
#12783=DIRECTION ( 'NONE',  ( -1.000000000000000000, 0.000000000000000000, 0.000000000000000000 ) ) ;
#12844=PRODUCT ( 'connector', 'connector', '', ( #14023 ) ) ;
#12917=ORIENTED_EDGE ( 'NONE', *, *, #639, .T. ) ;
#12943=VECTOR ( 'NONE', #14790, 1000.000000000000000 ) ;
#13016=EDGE_CURVE ( 'NONE', #3564, #6637, #1972, .T. ) ;
#13031=ORIENTED_EDGE ( 'NONE', *, *, #6676, .F. ) ;
#13111=DIRECTION ( 'NONE',  ( 1.000000000000000000, 0.000000000000000000, 0.000000000000000000 ) ) ;
#13112=CIRCLE ( 'NONE', #15162, 1.500000000000000000 ) ;
#13123=EDGE_CURVE ( 'NONE', #15509, #8237, #1213, .T. ) ;
#13162=CIRCLE ( 'NONE', #2747, 12.50000000000000533 ) ;
#13175=EDGE_LOOP ( 'NONE', ( #7791, #5558, #532, #14236 ) ) ;
#13248=CARTESIAN_POINT ( 'NONE',  ( 0.000000000000000000, 0.000000000000000000, 5.000000000000004441 ) ) ;
#13277=AXIS2_PLACEMENT_3D ( 'NONE', #10681, #15303, #15617 ) ;
#13278=FILL_AREA_STYLE_COLOUR ( '', #12537 ) ;
#13291=EDGE_CURVE ( 'NONE', #12484, #920, #13162, .T. ) ;
#13300=AXIS2_PLACEMENT_3D ( 'NONE', #9876, #6063, #10982 ) ;
#13306=CARTESIAN_POINT ( 'NONE',  ( -12.50000000000000533, 0.000000000000000000, 0.000000000000000000 ) ) ;
#13332=ORIENTED_EDGE ( 'NONE', *, *, #2651, .F. ) ;
#13353=CARTESIAN_POINT ( 'NONE',  ( -3.000000000000000000, 0.000000000000000000, 5.000000000000004441 ) ) ;
#13359=FACE_OUTER_BOUND ( 'NONE', #5340, .T. ) ;
#13395=CARTESIAN_POINT ( 'NONE',  ( -9.750000000000003553, 3.401296724241641415E-14, 0.000000000000000000 ) ) ;
#13435=VERTEX_POINT ( 'NONE', #3721 ) ;
#13442=DIRECTION ( 'NONE',  ( 1.000000000000000000, 0.000000000000000000, 0.000000000000000000 ) ) ;
#13470=EDGE_CURVE ( 'NONE', #6637, #3564, #15194, .T. ) ;
#13475=FACE_OUTER_BOUND ( 'NONE', #14569, .T. ) ;
#13496=DIRECTION ( 'NONE',  ( -1.000000000000000000, 0.000000000000000000, 0.000000000000000000 ) ) ;
#13501=PRODUCT_DEFINITION_SHAPE ( 'NONE', 'NONE',  #13615 ) ;
#13507=LINE ( 'NONE', #228, #15181 ) ;
#13512=CARTESIAN_POINT ( 'NONE',  ( 0.000000000000000000, 0.000000000000000000, 2.000000000000001776 ) ) ;
#13534=DIRECTION ( 'NONE',  ( 1.000000000000000000, 0.000000000000000000, 0.000000000000000000 ) ) ;
#13594=DIRECTION ( 'NONE',  ( -1.000000000000000000, 0.000000000000000000, 0.000000000000000000 ) ) ;
#13600=EDGE_LOOP ( 'NONE', ( #6407, #3680, #5727, #3599 ) ) ;
#13615=PRODUCT_DEFINITION ( 'UNKNOWN', '', #4771, #3074 ) ;
#13626=DIRECTION ( 'NONE',  ( 0.000000000000000000, 0.000000000000000000, 1.000000000000000000 ) ) ;
#13708=( GEOMETRIC_REPRESENTATION_CONTEXT ( 3 ) GLOBAL_UNCERTAINTY_ASSIGNED_CONTEXT ( ( #8404 ) ) GLOBAL_UNIT_ASSIGNED_CONTEXT ( ( #775, #8509, #14621 ) ) REPRESENTATION_CONTEXT ( 'NONE', 'WORKASPACE' ) );
#13806=VECTOR ( 'NONE', #1891, 1000.000000000000000 ) ;
#13858=DIRECTION ( 'NONE',  ( 0.000000000000000000, 0.000000000000000000, 1.000000000000000000 ) ) ;
#13862=CARTESIAN_POINT ( 'NONE',  ( 3.000000000000000000, 3.673940397442059868E-16, 5.000000000000004441 ) ) ;
#13950=VERTEX_POINT ( 'NONE', #7756 ) ;
#13970=EDGE_CURVE ( 'NONE', #13435, #1133, #15466, .T. ) ;
#14010=AXIS2_PLACEMENT_3D ( 'NONE', #7434, #9675, #1145 ) ;
#14023=PRODUCT_CONTEXT ( 'NONE', #9645, 'mechanical' ) ;
#14083=ORIENTED_EDGE ( 'NONE', *, *, #5221, .F. ) ;
#14102=ORIENTED_EDGE ( 'NONE', *, *, #7851, .T. ) ;
#14117=LINE ( 'NONE', #3377, #2919 ) ;
#14135=FACE_OUTER_BOUND ( 'NONE', #9957, .T. ) ;
#14136=AXIS2_PLACEMENT_3D ( 'NONE', #13248, #12053, #1152 ) ;
#14144=DIRECTION ( 'NONE',  ( 0.000000000000000000, 0.000000000000000000, 1.000000000000000000 ) ) ;
#14167=AXIS2_PLACEMENT_3D ( 'NONE', #12384, #6442, #6518 ) ;
#14201=AXIS2_PLACEMENT_3D ( 'NONE', #6680, #11513, #1651 ) ;
#14202=EDGE_CURVE ( 'NONE', #14655, #1178, #183, .T. ) ;
#14236=ORIENTED_EDGE ( 'NONE', *, *, #2004, .F. ) ;
#14267=DIRECTION ( 'NONE',  ( 1.000000000000000000, 0.000000000000000000, 0.000000000000000000 ) ) ;
#14349=CLOSED_SHELL ( 'NONE', ( #10212, #1823, #15565, #3854, #5372, #6826, #6651, #7081, #4849, #1622, #3267, #9338, #12644, #3814, #1519, #9461, #6599 ) ) ;
#14358=ORIENTED_EDGE ( 'NONE', *, *, #2498, .F. ) ;
#14381=EDGE_LOOP ( 'NONE', ( #10908, #3347 ) ) ;
#14431=DIRECTION ( 'NONE',  ( 1.000000000000000000, 0.000000000000000000, 0.000000000000000000 ) ) ;
#14445=CARTESIAN_POINT ( 'NONE',  ( -1.500000000000000000, 9.750000000000003553, 0.000000000000000000 ) ) ;
#14486=ORIENTED_EDGE ( 'NONE', *, *, #639, .F. ) ;
#14509=DIRECTION ( 'NONE',  ( 0.000000000000000000, 0.000000000000000000, 1.000000000000000000 ) ) ;
#14569=EDGE_LOOP ( 'NONE', ( #13031, #15432, #3587, #7411 ) ) ;
#14609=ORIENTED_EDGE ( 'NONE', *, *, #1432, .T. ) ;
#14611=CARTESIAN_POINT ( 'NONE',  ( 8.250000000000003553, -1.019131563299854308E-13, 2.000000000000001776 ) ) ;
#14621=( NAMED_UNIT ( * ) SI_UNIT ( $, .STERADIAN. ) SOLID_ANGLE_UNIT ( ) );
#14634=ORIENTED_EDGE ( 'NONE', *, *, #7181, .T. ) ;
#14641=DIRECTION ( 'NONE',  ( 0.000000000000000000, 0.000000000000000000, 1.000000000000000000 ) ) ;
#14644=CIRCLE ( 'NONE', #6774, 1.500000000000000000 ) ;
#14645=DIRECTION ( 'NONE',  ( 0.000000000000000000, 0.000000000000000000, 1.000000000000000000 ) ) ;
#14647=DIRECTION ( 'NONE',  ( 0.000000000000000000, 0.000000000000000000, 1.000000000000000000 ) ) ;
#14655=VERTEX_POINT ( 'NONE', #9804 ) ;
#14657=CARTESIAN_POINT ( 'NONE',  ( 0.000000000000000000, 0.000000000000000000, 5.000000000000004441 ) ) ;
#14689=DIRECTION ( 'NONE',  ( 0.000000000000000000, 0.000000000000000000, 1.000000000000000000 ) ) ;
#14721=FACE_BOUND ( 'NONE', #7277, .T. ) ;
#14726=CARTESIAN_POINT ( 'NONE',  ( 11.25000000000000355, -1.020968533498575335E-13, 0.000000000000000000 ) ) ;
#14730=EDGE_LOOP ( 'NONE', ( #7199, #1957 ) ) ;
#14743=( GEOMETRIC_REPRESENTATION_CONTEXT ( 3 ) GLOBAL_UNCERTAINTY_ASSIGNED_CONTEXT ( ( #2333 ) ) GLOBAL_UNIT_ASSIGNED_CONTEXT ( ( #8736, #9697, #288 ) ) REPRESENTATION_CONTEXT ( 'NONE', 'WORKASPACE' ) );
#14790=DIRECTION ( 'NONE',  ( 0.000000000000000000, 0.000000000000000000, -1.000000000000000000 ) ) ;
#14806=ORIENTED_EDGE ( 'NONE', *, *, #9648, .T. ) ;
#14866=DIRECTION ( 'NONE',  ( 1.000000000000000000, 0.000000000000000000, 0.000000000000000000 ) ) ;
#14889=CIRCLE ( 'NONE', #5738, 3.000000000000000000 ) ;
#14960=CIRCLE ( 'NONE', #2770, 3.000000000000000000 ) ;
#14965=CARTESIAN_POINT ( 'NONE',  ( 0.000000000000000000, 0.000000000000000000, 2.000000000000001776 ) ) ;
#15025=ORIENTED_EDGE ( 'NONE', *, *, #13123, .F. ) ;
#15041=ORIENTED_EDGE ( 'NONE', *, *, #2004, .T. ) ;
#15064=CARTESIAN_POINT ( 'NONE',  ( -3.000000000000000000, 0.000000000000000000, 5.000000000000004441 ) ) ;
#15102=ORIENTED_EDGE ( 'NONE', *, *, #7218, .F. ) ;
#15129=DIRECTION ( 'NONE',  ( 0.000000000000000000, 0.000000000000000000, 1.000000000000000000 ) ) ;
#15130=CIRCLE ( 'NONE', #10057, 1.499999999999999556 ) ;
#15136=VERTEX_POINT ( 'NONE', #282 ) ;
#15162=AXIS2_PLACEMENT_3D ( 'NONE', #6825, #11661, #6904 ) ;
#15178=CYLINDRICAL_SURFACE ( 'NONE', #4322, 1.500000000000000000 ) ;
#15181=VECTOR ( 'NONE', #304, 1000.000000000000000 ) ;
#15187=CYLINDRICAL_SURFACE ( 'NONE', #11359, 12.50000000000000533 ) ;
#15194=CIRCLE ( 'NONE', #3004, 5.000000000000000000 ) ;
#15211=EDGE_LOOP ( 'NONE', ( #2114, #1740, #9007, #3044 ) ) ;
#15285=DIRECTION ( 'NONE',  ( 1.000000000000000000, 0.000000000000000000, 0.000000000000000000 ) ) ;
#15303=DIRECTION ( 'NONE',  ( 0.000000000000000000, 0.000000000000000000, 1.000000000000000000 ) ) ;
#15335=CARTESIAN_POINT ( 'NONE',  ( 5.000000000000000000, 6.123233995736766282E-16, 5.000000000000004441 ) ) ;
#15336=ORIENTED_EDGE ( 'NONE', *, *, #10673, .F. ) ;
#15339=CARTESIAN_POINT ( 'NONE',  ( -9.750000000000003553, 3.401296724241641415E-14, 2.000000000000001776 ) ) ;
#15425=CARTESIAN_POINT ( 'NONE',  ( -1.500000000000000000, -9.750000000000003553, 2.000000000000001776 ) ) ;
#15432=ORIENTED_EDGE ( 'NONE', *, *, #11511, .T. ) ;
#15466=CIRCLE ( 'NONE', #8354, 1.499999999999999556 ) ;
#15483=DIRECTION ( 'NONE',  ( 0.000000000000000000, 0.000000000000000000, 1.000000000000000000 ) ) ;
#15509=VERTEX_POINT ( 'NONE', #15064 ) ;
#15565=ADVANCED_FACE ( 'NONE', ( #8797 ), #8040, .F. ) ;
#15592=VECTOR ( 'NONE', #14645, 1000.000000000000000 ) ;
#15617=DIRECTION ( 'NONE',  ( 1.000000000000000000, 0.000000000000000000, 0.000000000000000000 ) ) ;
#15623=ORIENTED_EDGE ( 'NONE', *, *, #11739, .T. ) ;
#15665=ORIENTED_EDGE ( 'NONE', *, *, #7781, .F. ) ;
#15673=DIRECTION ( 'NONE',  ( 0.000000000000000000, 0.000000000000000000, -1.000000000000000000 ) ) ;
#15686=AXIS2_PLACEMENT_3D ( 'NONE', #7309, #1248, #6123 ) ;
#15709=VERTEX_POINT ( 'NONE', #10254 ) ;
ENDSEC;
END-ISO-10303-21;
